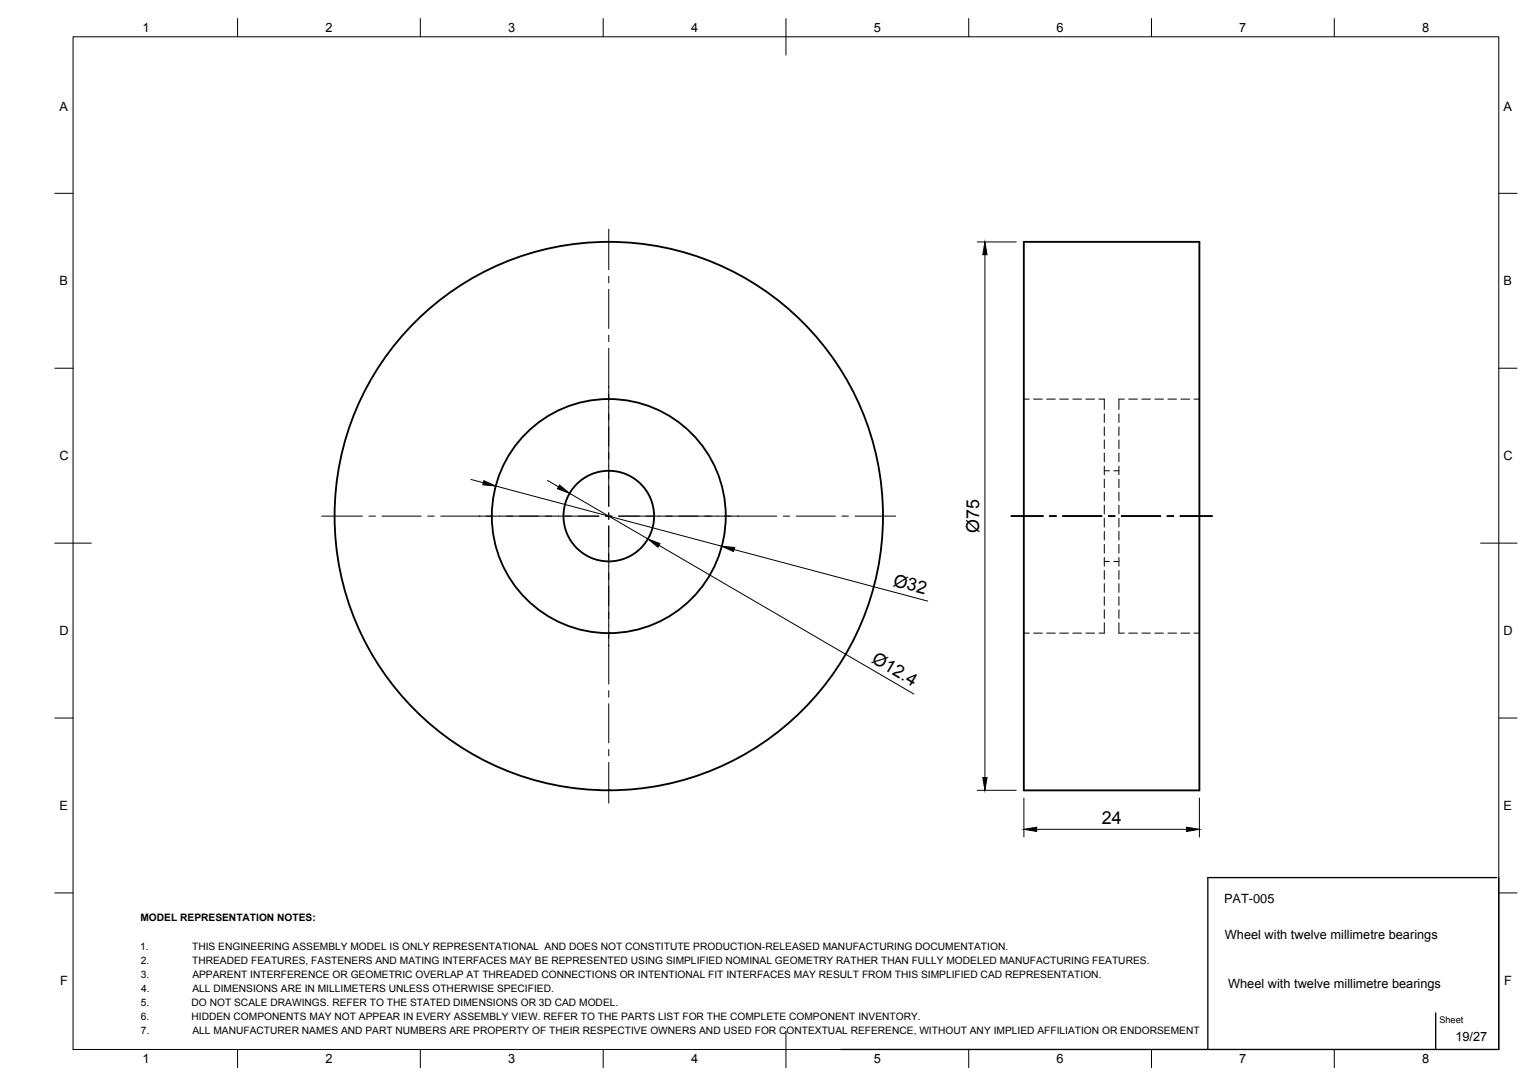
ISO-10303-21;
HEADER;
/* Generated by software containing ST-Developer
 * from STEP Tools, Inc. (www.steptools.com) 
 */

FILE_DESCRIPTION(
/* description */ ('Ball-race swivel caster'),
/* implementation_level */ '2;1');

FILE_NAME(
/* name */ 'Wheel with twelve millimetre bearings.step',
/* time_stamp */ '2026-10-29T16:15:51-07:00',
/* author */ (''),
/* organization */ (''),
/* preprocessor_version */ 'ST-DEVELOPER v20.2',
/* originating_system */ 'Autodesk Translation Framework v15.17.0.0',
/* authorisation */ '');

FILE_SCHEMA (('AUTOMOTIVE_DESIGN { 1 0 10303 214 3 1 1 }'));
ENDSEC;

DATA;
#10=MECHANICAL_DESIGN_GEOMETRIC_PRESENTATION_REPRESENTATION('',(#320),#7816);
#271=SHAPE_REPRESENTATION_RELATIONSHIP('SRR','None',#7919,#291);
#291=ADVANCED_BREP_SHAPE_REPRESENTATION('',(#355),#7808);
#320=STYLED_ITEM('',(#8097),#355);
#355=MANIFOLD_SOLID_BREP('Body1',#3727);
#423=FACE_BOUND('',#938,.T.);
#424=FACE_BOUND('',#941,.T.);
#425=FACE_BOUND('',#945,.T.);
#426=FACE_BOUND('',#947,.T.);
#502=PLANE('',#4331);
#503=PLANE('',#4336);
#504=PLANE('',#4342);
#505=PLANE('',#4343);
#673=FACE_OUTER_BOUND('',#936,.T.);
#674=FACE_OUTER_BOUND('',#937,.T.);
#675=FACE_OUTER_BOUND('',#939,.T.);
#676=FACE_OUTER_BOUND('',#940,.T.);
#677=FACE_OUTER_BOUND('',#942,.T.);
#678=FACE_OUTER_BOUND('',#943,.T.);
#679=FACE_OUTER_BOUND('',#944,.T.);
#680=FACE_OUTER_BOUND('',#946,.T.);
#936=EDGE_LOOP('',(#3193,#3194,#3195,#3196));
#937=EDGE_LOOP('',(#3197));
#938=EDGE_LOOP('',(#3198));
#939=EDGE_LOOP('',(#3199,#3200,#3201,#3202));
#940=EDGE_LOOP('',(#3203));
#941=EDGE_LOOP('',(#3204));
#942=EDGE_LOOP('',(#3205,#3206,#3207,#3208));
#943=EDGE_LOOP('',(#3209,#3210,#3211,#3212));
#944=EDGE_LOOP('',(#3213));
#945=EDGE_LOOP('',(#3214));
#946=EDGE_LOOP('',(#3215));
#947=EDGE_LOOP('',(#3216));
#1144=LINE('',#7190,#1299);
#1145=LINE('',#7199,#1300);
#1146=LINE('',#7205,#1301);
#1147=LINE('',#7210,#1302);
#1299=VECTOR('',#5358,1.6);
#1300=VECTOR('',#5369,1.6);
#1301=VECTOR('',#5378,0.62);
#1302=VECTOR('',#5383,3.75);
#1504=CIRCLE('',#4329,1.6);
#1505=CIRCLE('',#4330,1.6);
#1506=CIRCLE('',#4332,0.62);
#1507=CIRCLE('',#4334,1.6);
#1508=CIRCLE('',#4335,1.6);
#1509=CIRCLE('',#4337,0.62);
#1510=CIRCLE('',#4340,3.75);
#1511=CIRCLE('',#4341,3.75);
#1850=VERTEX_POINT('',#7187);
#1851=VERTEX_POINT('',#7189);
#1852=VERTEX_POINT('',#7193);
#1853=VERTEX_POINT('',#7196);
#1854=VERTEX_POINT('',#7198);
#1855=VERTEX_POINT('',#7202);
#1856=VERTEX_POINT('',#7207);
#1857=VERTEX_POINT('',#7209);
#2316=EDGE_CURVE('',#1850,#1850,#1504,.T.);
#2317=EDGE_CURVE('',#1850,#1851,#1144,.T.);
#2318=EDGE_CURVE('',#1851,#1851,#1505,.T.);
#2319=EDGE_CURVE('',#1852,#1852,#1506,.T.);
#2320=EDGE_CURVE('',#1853,#1853,#1507,.T.);
#2321=EDGE_CURVE('',#1853,#1854,#1145,.T.);
#2322=EDGE_CURVE('',#1854,#1854,#1508,.T.);
#2323=EDGE_CURVE('',#1855,#1855,#1509,.T.);
#2324=EDGE_CURVE('',#1855,#1852,#1146,.T.);
#2325=EDGE_CURVE('',#1856,#1856,#1510,.T.);
#2326=EDGE_CURVE('',#1856,#1857,#1147,.T.);
#2327=EDGE_CURVE('',#1857,#1857,#1511,.T.);
#3193=ORIENTED_EDGE('',*,*,#2316,.F.);
#3194=ORIENTED_EDGE('',*,*,#2317,.T.);
#3195=ORIENTED_EDGE('',*,*,#2318,.F.);
#3196=ORIENTED_EDGE('',*,*,#2317,.F.);
#3197=ORIENTED_EDGE('',*,*,#2316,.T.);
#3198=ORIENTED_EDGE('',*,*,#2319,.F.);
#3199=ORIENTED_EDGE('',*,*,#2320,.F.);
#3200=ORIENTED_EDGE('',*,*,#2321,.T.);
#3201=ORIENTED_EDGE('',*,*,#2322,.T.);
#3202=ORIENTED_EDGE('',*,*,#2321,.F.);
#3203=ORIENTED_EDGE('',*,*,#2322,.F.);
#3204=ORIENTED_EDGE('',*,*,#2323,.F.);
#3205=ORIENTED_EDGE('',*,*,#2323,.T.);
#3206=ORIENTED_EDGE('',*,*,#2324,.T.);
#3207=ORIENTED_EDGE('',*,*,#2319,.T.);
#3208=ORIENTED_EDGE('',*,*,#2324,.F.);
#3209=ORIENTED_EDGE('',*,*,#2325,.F.);
#3210=ORIENTED_EDGE('',*,*,#2326,.T.);
#3211=ORIENTED_EDGE('',*,*,#2327,.T.);
#3212=ORIENTED_EDGE('',*,*,#2326,.F.);
#3213=ORIENTED_EDGE('',*,*,#2325,.T.);
#3214=ORIENTED_EDGE('',*,*,#2318,.T.);
#3215=ORIENTED_EDGE('',*,*,#2327,.F.);
#3216=ORIENTED_EDGE('',*,*,#2320,.T.);
#3477=CYLINDRICAL_SURFACE('',#4328,1.6);
#3478=CYLINDRICAL_SURFACE('',#4333,1.6);
#3479=CYLINDRICAL_SURFACE('',#4338,0.62);
#3480=CYLINDRICAL_SURFACE('',#4339,3.75);
#3644=ADVANCED_FACE('',(#673),#3477,.F.);
#3645=ADVANCED_FACE('',(#674,#423),#502,.T.);
#3646=ADVANCED_FACE('',(#675),#3478,.F.);
#3647=ADVANCED_FACE('',(#676,#424),#503,.F.);
#3648=ADVANCED_FACE('',(#677),#3479,.F.);
#3649=ADVANCED_FACE('',(#678),#3480,.T.);
#3650=ADVANCED_FACE('',(#679,#425),#504,.T.);
#3651=ADVANCED_FACE('',(#680,#426),#505,.F.);
#3727=CLOSED_SHELL('',(#3644,#3645,#3646,#3647,#3648,#3649,#3650,#3651));
#4327=AXIS2_PLACEMENT_3D('',#7185,#5352,#5353);
#4328=AXIS2_PLACEMENT_3D('',#7186,#5354,#5355);
#4329=AXIS2_PLACEMENT_3D('',#7188,#5356,#5357);
#4330=AXIS2_PLACEMENT_3D('',#7191,#5359,#5360);
#4331=AXIS2_PLACEMENT_3D('',#7192,#5361,#5362);
#4332=AXIS2_PLACEMENT_3D('',#7194,#5363,#5364);
#4333=AXIS2_PLACEMENT_3D('',#7195,#5365,#5366);
#4334=AXIS2_PLACEMENT_3D('',#7197,#5367,#5368);
#4335=AXIS2_PLACEMENT_3D('',#7200,#5370,#5371);
#4336=AXIS2_PLACEMENT_3D('',#7201,#5372,#5373);
#4337=AXIS2_PLACEMENT_3D('',#7203,#5374,#5375);
#4338=AXIS2_PLACEMENT_3D('',#7204,#5376,#5377);
#4339=AXIS2_PLACEMENT_3D('',#7206,#5379,#5380);
#4340=AXIS2_PLACEMENT_3D('',#7208,#5381,#5382);
#4341=AXIS2_PLACEMENT_3D('',#7211,#5384,#5385);
#4342=AXIS2_PLACEMENT_3D('',#7212,#5386,#5387);
#4343=AXIS2_PLACEMENT_3D('',#7213,#5388,#5389);
#5352=DIRECTION('axis',(0.,0.,1.));
#5353=DIRECTION('refdir',(1.,0.,0.));
#5354=DIRECTION('center_axis',(0.,1.,0.));
#5355=DIRECTION('ref_axis',(1.,0.,0.));
#5356=DIRECTION('center_axis',(0.,1.,0.));
#5357=DIRECTION('ref_axis',(1.,0.,0.));
#5358=DIRECTION('',(0.,1.,0.));
#5359=DIRECTION('center_axis',(0.,-1.,0.));
#5360=DIRECTION('ref_axis',(1.,0.,0.));
#5361=DIRECTION('center_axis',(0.,1.,0.));
#5362=DIRECTION('ref_axis',(1.,0.,0.));
#5363=DIRECTION('center_axis',(0.,1.,0.));
#5364=DIRECTION('ref_axis',(1.,0.,0.));
#5365=DIRECTION('center_axis',(0.,1.,0.));
#5366=DIRECTION('ref_axis',(1.,0.,0.));
#5367=DIRECTION('center_axis',(0.,1.,0.));
#5368=DIRECTION('ref_axis',(1.,0.,0.));
#5369=DIRECTION('',(0.,1.,0.));
#5370=DIRECTION('center_axis',(0.,1.,0.));
#5371=DIRECTION('ref_axis',(1.,0.,0.));
#5372=DIRECTION('center_axis',(0.,1.,0.));
#5373=DIRECTION('ref_axis',(1.,0.,0.));
#5374=DIRECTION('center_axis',(0.,-1.,0.));
#5375=DIRECTION('ref_axis',(1.,0.,0.));
#5376=DIRECTION('center_axis',(0.,1.,0.));
#5377=DIRECTION('ref_axis',(1.,0.,0.));
#5378=DIRECTION('',(0.,1.,0.));
#5379=DIRECTION('center_axis',(0.,1.,0.));
#5380=DIRECTION('ref_axis',(1.,0.,0.));
#5381=DIRECTION('center_axis',(0.,1.,0.));
#5382=DIRECTION('ref_axis',(1.,0.,0.));
#5383=DIRECTION('',(0.,-1.,0.));
#5384=DIRECTION('center_axis',(0.,1.,0.));
#5385=DIRECTION('ref_axis',(1.,0.,0.));
#5386=DIRECTION('center_axis',(0.,1.,0.));
#5387=DIRECTION('ref_axis',(1.,0.,0.));
#5388=DIRECTION('center_axis',(0.,1.,0.));
#5389=DIRECTION('ref_axis',(1.,0.,0.));
#7185=CARTESIAN_POINT('',(0.,0.,0.));
#7186=CARTESIAN_POINT('Origin',(0.,0.1,4.));
#7187=CARTESIAN_POINT('',(-1.6,0.1,4.));
#7188=CARTESIAN_POINT('Origin',(0.,0.1,4.));
#7189=CARTESIAN_POINT('',(-1.6,1.2,4.));
#7190=CARTESIAN_POINT('',(-1.6,0.1,4.));
#7191=CARTESIAN_POINT('Origin',(0.,1.2,4.));
#7192=CARTESIAN_POINT('Origin',(0.,0.1,4.));
#7193=CARTESIAN_POINT('',(-0.62,0.1,4.));
#7194=CARTESIAN_POINT('Origin',(0.,0.1,4.));
#7195=CARTESIAN_POINT('Origin',(0.,-1.3,4.));
#7196=CARTESIAN_POINT('',(-1.6,-1.2,4.));
#7197=CARTESIAN_POINT('Origin',(0.,-1.2,4.));
#7198=CARTESIAN_POINT('',(-1.6,-0.0999999999999999,4.));
#7199=CARTESIAN_POINT('',(-1.6,-1.3,4.));
#7200=CARTESIAN_POINT('Origin',(0.,-0.0999999999999999,4.));
#7201=CARTESIAN_POINT('Origin',(0.,-0.0999999999999999,4.));
#7202=CARTESIAN_POINT('',(-0.62,-0.0999999999999999,4.));
#7203=CARTESIAN_POINT('Origin',(0.,-0.0999999999999999,4.));
#7204=CARTESIAN_POINT('Origin',(0.,-1.3,4.));
#7205=CARTESIAN_POINT('',(-0.62,-1.3,4.));
#7206=CARTESIAN_POINT('Origin',(0.,-1.2,4.));
#7207=CARTESIAN_POINT('',(-3.75,1.2,4.));
#7208=CARTESIAN_POINT('Origin',(0.,1.2,4.));
#7209=CARTESIAN_POINT('',(-3.75,-1.2,4.));
#7210=CARTESIAN_POINT('',(-3.75,-1.2,4.));
#7211=CARTESIAN_POINT('Origin',(0.,-1.2,4.));
#7212=CARTESIAN_POINT('Origin',(0.,1.2,4.));
#7213=CARTESIAN_POINT('Origin',(0.,-1.2,4.));
#7781=UNCERTAINTY_MEASURE_WITH_UNIT(LENGTH_MEASURE(0.001),#7817,
'DISTANCE_ACCURACY_VALUE',
'Maximum model space distance between geometric entities at asserted c
onnectivities');
#7789=UNCERTAINTY_MEASURE_WITH_UNIT(LENGTH_MEASURE(0.001),#7817,
'DISTANCE_ACCURACY_VALUE',
'Maximum model space distance between geometric entities at asserted c
onnectivities');
#7808=(
GEOMETRIC_REPRESENTATION_CONTEXT(3)
GLOBAL_UNCERTAINTY_ASSIGNED_CONTEXT((#7781))
GLOBAL_UNIT_ASSIGNED_CONTEXT((#7817,#7819,#7820))
REPRESENTATION_CONTEXT('','3D')
);
#7816=(
GEOMETRIC_REPRESENTATION_CONTEXT(3)
GLOBAL_UNCERTAINTY_ASSIGNED_CONTEXT((#7789))
GLOBAL_UNIT_ASSIGNED_CONTEXT((#7817,#7819,#7820))
REPRESENTATION_CONTEXT('','3D')
);
#7817=(
LENGTH_UNIT()
NAMED_UNIT(*)
SI_UNIT(.CENTI.,.METRE.)
);
#7819=(
NAMED_UNIT(*)
PLANE_ANGLE_UNIT()
SI_UNIT($,.RADIAN.)
);
#7820=(
NAMED_UNIT(*)
SI_UNIT($,.STERADIAN.)
SOLID_ANGLE_UNIT()
);
#7839=SHAPE_DEFINITION_REPRESENTATION(#7880,#7919);
#7880=PRODUCT_DEFINITION_SHAPE('',$,#7946);
#7919=SHAPE_REPRESENTATION('',(#4327),#7808);
#7927=PRODUCT_DEFINITION_CONTEXT('part definition',#8007,'design');
#7946=PRODUCT_DEFINITION('Wheel with twelve millimetre bearings',
'Wheel with twelve millimetre bearings',#7972,#7927);
#7972=PRODUCT_DEFINITION_FORMATION('',$,#8027);
#8007=APPLICATION_CONTEXT(
'Core Data for Automotive Mechanical Design Process');
#8008=PRODUCT_CONTEXT('part definition',#8007,'mechanical');
#8027=PRODUCT('Wheel with twelve millimetre bearings',
'Wheel with twelve millimetre bearings',
'Wheel with twelve millimetre bearings',(#8008));
#8091=COLOUR_RGB('Grey',0.48,0.52,0.57);
#8092=FILL_AREA_STYLE_COLOUR('',#8091);
#8093=FILL_AREA_STYLE('',(#8092));
#8094=SURFACE_STYLE_FILL_AREA(#8093);
#8095=SURFACE_SIDE_STYLE('',(#8094));
#8096=SURFACE_STYLE_USAGE(.BOTH.,#8095);
#8097=PRESENTATION_STYLE_ASSIGNMENT((#8096));
ENDSEC;
END-ISO-10303-21;
